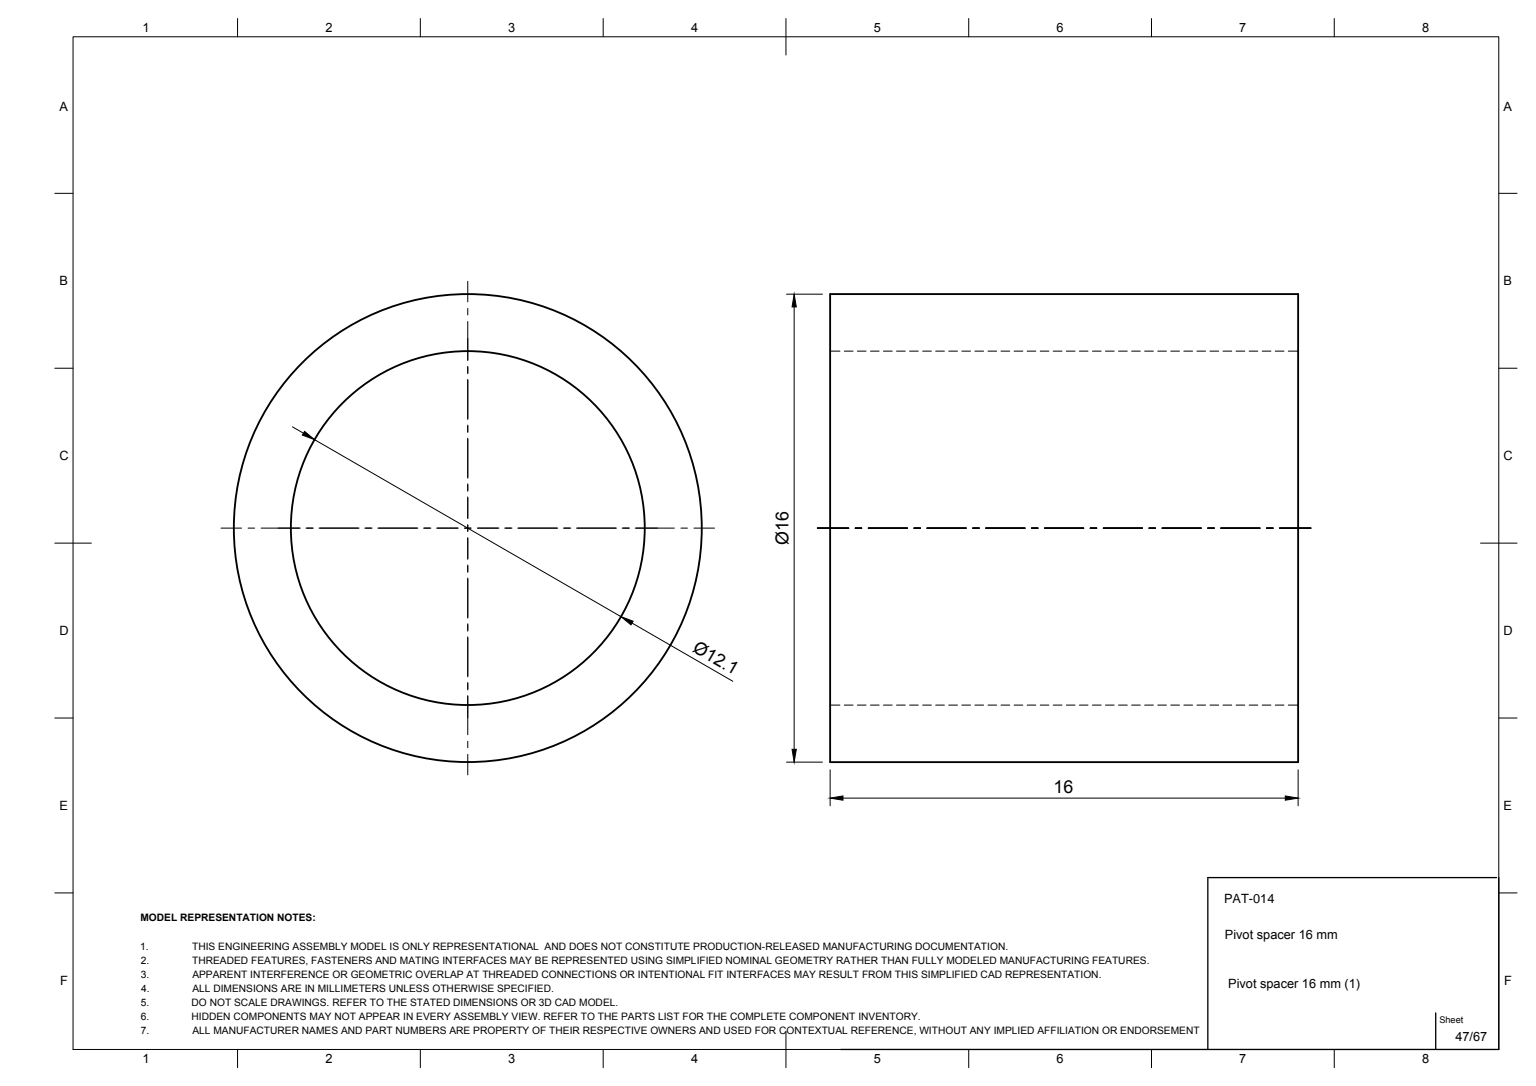
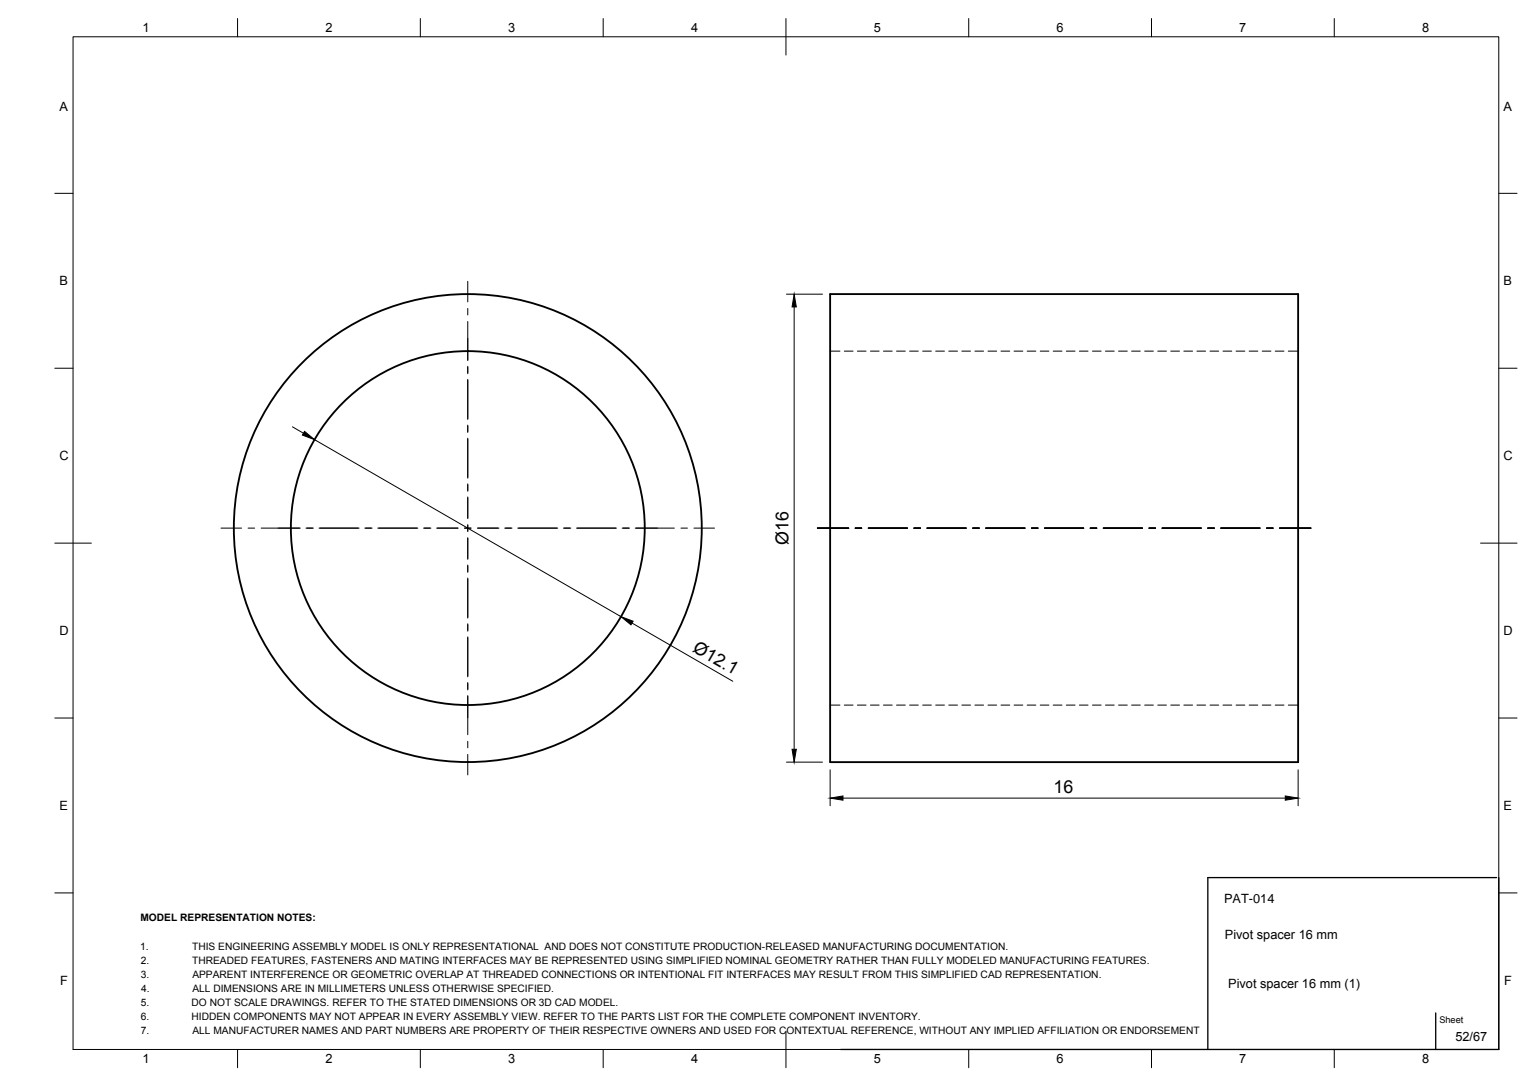
ISO-10303-21;
HEADER;
/* Generated by software containing ST-Developer
 * from STEP Tools, Inc. (www.steptools.com) 
 */

FILE_DESCRIPTION(
/* description */ ('Bin tilter linkage'),
/* implementation_level */ '2;1');

FILE_NAME(
/* name */ 'Pivot spacer 16 mm (1).step',
/* time_stamp */ '2026-10-28T03:26:24-07:00',
/* author */ (''),
/* organization */ (''),
/* preprocessor_version */ 'ST-DEVELOPER v20.2',
/* originating_system */ 'Autodesk Translation Framework v15.17.0.0',
/* authorisation */ '');

FILE_SCHEMA (('AUTOMOTIVE_DESIGN { 1 0 10303 214 3 1 1 }'));
ENDSEC;

DATA;
#10=MECHANICAL_DESIGN_GEOMETRIC_PRESENTATION_REPRESENTATION('',(#956),#23728);
#736=SHAPE_REPRESENTATION_RELATIONSHIP('SRR','None',#24204,#842);
#842=ADVANCED_BREP_SHAPE_REPRESENTATION('',(#1069),#23704);
#956=STYLED_ITEM('',(#24779),#1069);
#1069=MANIFOLD_SOLID_BREP('Body1',#12487);
#1437=FACE_BOUND('',#3652,.T.);
#1438=FACE_BOUND('',#3654,.T.);
#1799=PLANE('',#15109);
#1800=PLANE('',#15110);
#2522=FACE_OUTER_BOUND('',#3649,.T.);
#2523=FACE_OUTER_BOUND('',#3650,.T.);
#2524=FACE_OUTER_BOUND('',#3651,.T.);
#2525=FACE_OUTER_BOUND('',#3653,.T.);
#3649=EDGE_LOOP('',(#10729,#10730,#10731,#10732));
#3650=EDGE_LOOP('',(#10733,#10734,#10735,#10736));
#3651=EDGE_LOOP('',(#10737));
#3652=EDGE_LOOP('',(#10738));
#3653=EDGE_LOOP('',(#10739));
#3654=EDGE_LOOP('',(#10740));
#4362=LINE('',#22789,#5037);
#4363=LINE('',#22795,#5038);
#5037=VECTOR('',#18845,0.605);
#5038=VECTOR('',#18852,0.800000000000001);
#5850=CIRCLE('',#15104,0.605);
#5851=CIRCLE('',#15105,0.605);
#5852=CIRCLE('',#15107,0.800000000000001);
#5853=CIRCLE('',#15108,0.800000000000001);
#6749=VERTEX_POINT('',#22786);
#6750=VERTEX_POINT('',#22788);
#6751=VERTEX_POINT('',#22792);
#6752=VERTEX_POINT('',#22794);
#8104=EDGE_CURVE('',#6749,#6749,#5850,.T.);
#8105=EDGE_CURVE('',#6749,#6750,#4362,.T.);
#8106=EDGE_CURVE('',#6750,#6750,#5851,.T.);
#8107=EDGE_CURVE('',#6751,#6751,#5852,.T.);
#8108=EDGE_CURVE('',#6751,#6752,#4363,.T.);
#8109=EDGE_CURVE('',#6752,#6752,#5853,.T.);
#10729=ORIENTED_EDGE('',*,*,#8104,.F.);
#10730=ORIENTED_EDGE('',*,*,#8105,.T.);
#10731=ORIENTED_EDGE('',*,*,#8106,.T.);
#10732=ORIENTED_EDGE('',*,*,#8105,.F.);
#10733=ORIENTED_EDGE('',*,*,#8107,.F.);
#10734=ORIENTED_EDGE('',*,*,#8108,.T.);
#10735=ORIENTED_EDGE('',*,*,#8109,.T.);
#10736=ORIENTED_EDGE('',*,*,#8108,.F.);
#10737=ORIENTED_EDGE('',*,*,#8107,.T.);
#10738=ORIENTED_EDGE('',*,*,#8104,.T.);
#10739=ORIENTED_EDGE('',*,*,#8109,.F.);
#10740=ORIENTED_EDGE('',*,*,#8106,.F.);
#11568=CYLINDRICAL_SURFACE('',#15103,0.605);
#11569=CYLINDRICAL_SURFACE('',#15106,0.800000000000001);
#12247=ADVANCED_FACE('',(#2522),#11568,.F.);
#12248=ADVANCED_FACE('',(#2523),#11569,.T.);
#12249=ADVANCED_FACE('',(#2524,#1437),#1799,.T.);
#12250=ADVANCED_FACE('',(#2525,#1438),#1800,.F.);
#12487=CLOSED_SHELL('',(#12247,#12248,#12249,#12250));
#15102=AXIS2_PLACEMENT_3D('',#22784,#18839,#18840);
#15103=AXIS2_PLACEMENT_3D('',#22785,#18841,#18842);
#15104=AXIS2_PLACEMENT_3D('',#22787,#18843,#18844);
#15105=AXIS2_PLACEMENT_3D('',#22790,#18846,#18847);
#15106=AXIS2_PLACEMENT_3D('',#22791,#18848,#18849);
#15107=AXIS2_PLACEMENT_3D('',#22793,#18850,#18851);
#15108=AXIS2_PLACEMENT_3D('',#22796,#18853,#18854);
#15109=AXIS2_PLACEMENT_3D('',#22797,#18855,#18856);
#15110=AXIS2_PLACEMENT_3D('',#22798,#18857,#18858);
#18839=DIRECTION('axis',(0.,0.,1.));
#18840=DIRECTION('refdir',(1.,0.,0.));
#18841=DIRECTION('center_axis',(0.,1.,0.));
#18842=DIRECTION('ref_axis',(1.,0.,0.));
#18843=DIRECTION('center_axis',(0.,-1.,0.));
#18844=DIRECTION('ref_axis',(1.,0.,0.));
#18845=DIRECTION('',(0.,-1.,0.));
#18846=DIRECTION('center_axis',(0.,-1.,0.));
#18847=DIRECTION('ref_axis',(1.,0.,0.));
#18848=DIRECTION('center_axis',(0.,1.,0.));
#18849=DIRECTION('ref_axis',(1.,0.,0.));
#18850=DIRECTION('center_axis',(0.,1.,0.));
#18851=DIRECTION('ref_axis',(1.,0.,0.));
#18852=DIRECTION('',(0.,-1.,0.));
#18853=DIRECTION('center_axis',(0.,1.,0.));
#18854=DIRECTION('ref_axis',(1.,0.,0.));
#18855=DIRECTION('center_axis',(0.,1.,0.));
#18856=DIRECTION('ref_axis',(1.,0.,0.));
#18857=DIRECTION('center_axis',(0.,1.,0.));
#18858=DIRECTION('ref_axis',(1.,0.,0.));
#22784=CARTESIAN_POINT('',(0.,0.,0.));
#22785=CARTESIAN_POINT('Origin',(24.2020784790221,0.5,28.6577532024872));
#22786=CARTESIAN_POINT('',(23.5970784790221,2.1,28.6577532024872));
#22787=CARTESIAN_POINT('Origin',(24.2020784790221,2.1,28.6577532024872));
#22788=CARTESIAN_POINT('',(23.5970784790221,0.5,28.6577532024872));
#22789=CARTESIAN_POINT('',(23.5970784790221,0.5,28.6577532024872));
#22790=CARTESIAN_POINT('Origin',(24.2020784790221,0.5,28.6577532024872));
#22791=CARTESIAN_POINT('Origin',(24.2020784790221,0.5,28.6577532024872));
#22792=CARTESIAN_POINT('',(23.4020784790221,2.1,28.6577532024872));
#22793=CARTESIAN_POINT('Origin',(24.2020784790221,2.1,28.6577532024872));
#22794=CARTESIAN_POINT('',(23.4020784790221,0.5,28.6577532024872));
#22795=CARTESIAN_POINT('',(23.4020784790221,0.5,28.6577532024872));
#22796=CARTESIAN_POINT('Origin',(24.2020784790221,0.5,28.6577532024872));
#22797=CARTESIAN_POINT('Origin',(24.2020784790221,2.1,28.6577532024872));
#22798=CARTESIAN_POINT('Origin',(24.2020784790221,0.5,28.6577532024872));
#23587=UNCERTAINTY_MEASURE_WITH_UNIT(LENGTH_MEASURE(0.001),#23729,
'DISTANCE_ACCURACY_VALUE',
'Maximum model space distance between geometric entities at asserted c
onnectivities');
#23611=UNCERTAINTY_MEASURE_WITH_UNIT(LENGTH_MEASURE(0.001),#23729,
'DISTANCE_ACCURACY_VALUE',
'Maximum model space distance between geometric entities at asserted c
onnectivities');
#23704=(
GEOMETRIC_REPRESENTATION_CONTEXT(3)
GLOBAL_UNCERTAINTY_ASSIGNED_CONTEXT((#23587))
GLOBAL_UNIT_ASSIGNED_CONTEXT((#23729,#23731,#23732))
REPRESENTATION_CONTEXT('','3D')
);
#23728=(
GEOMETRIC_REPRESENTATION_CONTEXT(3)
GLOBAL_UNCERTAINTY_ASSIGNED_CONTEXT((#23611))
GLOBAL_UNIT_ASSIGNED_CONTEXT((#23729,#23731,#23732))
REPRESENTATION_CONTEXT('','3D')
);
#23729=(
LENGTH_UNIT()
NAMED_UNIT(*)
SI_UNIT(.CENTI.,.METRE.)
);
#23731=(
NAMED_UNIT(*)
PLANE_ANGLE_UNIT()
SI_UNIT($,.RADIAN.)
);
#23732=(
NAMED_UNIT(*)
SI_UNIT($,.STERADIAN.)
SOLID_ANGLE_UNIT()
);
#23825=SHAPE_DEFINITION_REPRESENTATION(#23992,#24204);
#23992=PRODUCT_DEFINITION_SHAPE('',$,#24321);
#24204=SHAPE_REPRESENTATION('',(#15102),#23704);
#24228=PRODUCT_DEFINITION_CONTEXT('part definition',#24578,'design');
#24321=PRODUCT_DEFINITION('Pivot spacer 16 mm (1)',
'Pivot spacer 16 mm (1)',#24437,#24228);
#24437=PRODUCT_DEFINITION_FORMATION('',$,#24672);
#24578=APPLICATION_CONTEXT(
'Core Data for Automotive Mechanical Design Process');
#24579=PRODUCT_CONTEXT('part definition',#24578,'mechanical');
#24672=PRODUCT('Pivot spacer 16 mm (1)','Pivot spacer 16 mm (1)',
'Pivot spacer 16 mm (1)',(#24579));
#24773=COLOUR_RGB('Off White',0.89,0.88,0.83);
#24774=FILL_AREA_STYLE_COLOUR('',#24773);
#24775=FILL_AREA_STYLE('',(#24774));
#24776=SURFACE_STYLE_FILL_AREA(#24775);
#24777=SURFACE_SIDE_STYLE('',(#24776));
#24778=SURFACE_STYLE_USAGE(.BOTH.,#24777);
#24779=PRESENTATION_STYLE_ASSIGNMENT((#24778));
ENDSEC;
END-ISO-10303-21;
